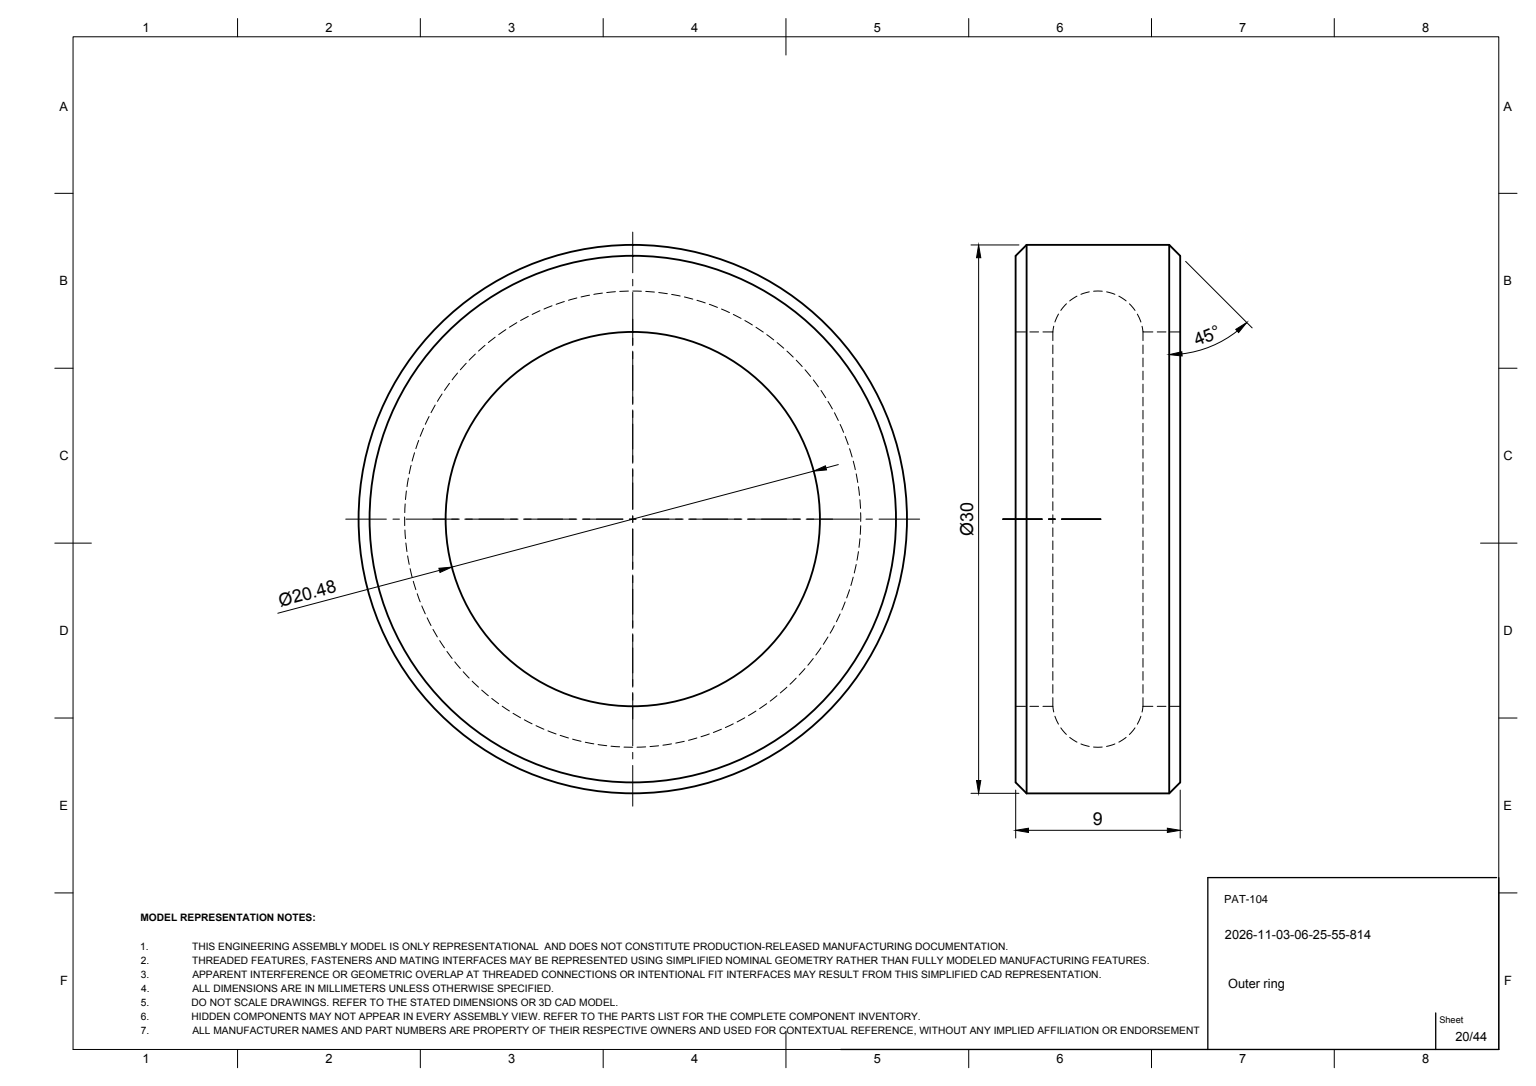
ISO-10303-21;
HEADER;
/* Generated by software containing ST-Developer
 * from STEP Tools, Inc. (www.steptools.com) 
 */

FILE_DESCRIPTION(
/* description */ ('Timing belt drive module 2 mm Pitch Timing 20T-40T'),

/* implementation_level */ '2;1');

FILE_NAME(
/* name */ 'Outer ring.step',
/* time_stamp */ '2026-10-28T03:25:12-07:00',
/* author */ (''),
/* organization */ (''),
/* preprocessor_version */ 'ST-DEVELOPER v20.2',
/* originating_system */ 'Autodesk Translation Framework v15.17.0.0',
/* authorisation */ '');

FILE_SCHEMA (('AUTOMOTIVE_DESIGN { 1 0 10303 214 3 1 1 }'));
ENDSEC;

DATA;
#10=MECHANICAL_DESIGN_GEOMETRIC_PRESENTATION_REPRESENTATION('',(#541),#17830);
#417=CONICAL_SURFACE('',#9909,1.47,0.785398163397449);
#418=CONICAL_SURFACE('',#9913,1.47,0.785398163397449);
#435=TOROIDAL_SURFACE('',#9898,1.,0.247676);
#455=SHAPE_REPRESENTATION_RELATIONSHIP('SRR','None',#18026,#498);
#498=ADVANCED_BREP_SHAPE_REPRESENTATION('',(#599),#17801);
#541=STYLED_ITEM('',(#18317),#599);
#599=MANIFOLD_SOLID_BREP('Body1',#8998);
#711=FACE_BOUND('',#1734,.T.);
#712=FACE_BOUND('',#1739,.T.);
#855=PLANE('',#9906);
#856=PLANE('',#9915);
#1136=FACE_OUTER_BOUND('',#1731,.T.);
#1137=FACE_OUTER_BOUND('',#1732,.T.);
#1138=FACE_OUTER_BOUND('',#1733,.T.);
#1139=FACE_OUTER_BOUND('',#1735,.T.);
#1140=FACE_OUTER_BOUND('',#1736,.T.);
#1141=FACE_OUTER_BOUND('',#1737,.T.);
#1142=FACE_OUTER_BOUND('',#1738,.T.);
#1143=FACE_OUTER_BOUND('',#1740,.T.);
#1731=EDGE_LOOP('',(#6573,#6574,#6575,#6576,#6577,#6578));
#1732=EDGE_LOOP('',(#6579,#6580,#6581,#6582,#6583));
#1733=EDGE_LOOP('',(#6584));
#1734=EDGE_LOOP('',(#6585));
#1735=EDGE_LOOP('',(#6586,#6587,#6588,#6589));
#1736=EDGE_LOOP('',(#6590,#6591,#6592,#6593));
#1737=EDGE_LOOP('',(#6594,#6595,#6596,#6597));
#1738=EDGE_LOOP('',(#6598));
#1739=EDGE_LOOP('',(#6599));
#1740=EDGE_LOOP('',(#6600,#6601,#6602,#6603,#6604));
#2327=CIRCLE('',#9899,1.023815);
#2328=CIRCLE('',#9900,1.023815);
#2329=CIRCLE('',#9901,0.247676);
#2330=CIRCLE('',#9902,1.023815);
#2331=CIRCLE('',#9903,1.023815);
#2332=CIRCLE('',#9905,1.023815);
#2333=CIRCLE('',#9907,1.44);
#2334=CIRCLE('',#9908,1.023815);
#2335=CIRCLE('',#9910,1.5);
#2336=CIRCLE('',#9912,1.5);
#2337=CIRCLE('',#9914,1.44);
#3003=LINE('',#14747,#3481);
#3004=LINE('',#14756,#3482);
#3005=LINE('',#14760,#3483);
#3006=LINE('',#14764,#3484);
#3007=LINE('',#14767,#3485);
#3481=VECTOR('',#11802,1.023815);
#3482=VECTOR('',#11813,1.47);
#3483=VECTOR('',#11818,1.5);
#3484=VECTOR('',#11823,1.47);
#3485=VECTOR('',#11828,1.023815);
#4012=VERTEX_POINT('',#14735);
#4013=VERTEX_POINT('',#14736);
#4014=VERTEX_POINT('',#14739);
#4015=VERTEX_POINT('',#14741);
#4016=VERTEX_POINT('',#14745);
#4017=VERTEX_POINT('',#14749);
#4018=VERTEX_POINT('',#14751);
#4019=VERTEX_POINT('',#14754);
#4020=VERTEX_POINT('',#14758);
#4021=VERTEX_POINT('',#14762);
#4969=EDGE_CURVE('',#4012,#4013,#2327,.T.);
#4970=EDGE_CURVE('',#4013,#4012,#2328,.T.);
#4971=EDGE_CURVE('',#4013,#4014,#2329,.T.);
#4972=EDGE_CURVE('',#4015,#4014,#2330,.T.);
#4973=EDGE_CURVE('',#4014,#4015,#2331,.T.);
#4974=EDGE_CURVE('',#4016,#4016,#2332,.T.);
#4975=EDGE_CURVE('',#4016,#4015,#3003,.T.);
#4976=EDGE_CURVE('',#4017,#4017,#2333,.T.);
#4977=EDGE_CURVE('',#4018,#4018,#2334,.T.);
#4978=EDGE_CURVE('',#4019,#4019,#2335,.T.);
#4979=EDGE_CURVE('',#4019,#4017,#3004,.T.);
#4980=EDGE_CURVE('',#4020,#4020,#2336,.T.);
#4981=EDGE_CURVE('',#4020,#4019,#3005,.T.);
#4982=EDGE_CURVE('',#4021,#4021,#2337,.T.);
#4983=EDGE_CURVE('',#4021,#4020,#3006,.T.);
#4984=EDGE_CURVE('',#4012,#4018,#3007,.T.);
#6573=ORIENTED_EDGE('',*,*,#4969,.F.);
#6574=ORIENTED_EDGE('',*,*,#4970,.F.);
#6575=ORIENTED_EDGE('',*,*,#4971,.T.);
#6576=ORIENTED_EDGE('',*,*,#4972,.F.);
#6577=ORIENTED_EDGE('',*,*,#4973,.F.);
#6578=ORIENTED_EDGE('',*,*,#4971,.F.);
#6579=ORIENTED_EDGE('',*,*,#4974,.T.);
#6580=ORIENTED_EDGE('',*,*,#4975,.T.);
#6581=ORIENTED_EDGE('',*,*,#4972,.T.);
#6582=ORIENTED_EDGE('',*,*,#4973,.T.);
#6583=ORIENTED_EDGE('',*,*,#4975,.F.);
#6584=ORIENTED_EDGE('',*,*,#4976,.F.);
#6585=ORIENTED_EDGE('',*,*,#4977,.T.);
#6586=ORIENTED_EDGE('',*,*,#4978,.F.);
#6587=ORIENTED_EDGE('',*,*,#4979,.T.);
#6588=ORIENTED_EDGE('',*,*,#4976,.T.);
#6589=ORIENTED_EDGE('',*,*,#4979,.F.);
#6590=ORIENTED_EDGE('',*,*,#4980,.F.);
#6591=ORIENTED_EDGE('',*,*,#4981,.T.);
#6592=ORIENTED_EDGE('',*,*,#4978,.T.);
#6593=ORIENTED_EDGE('',*,*,#4981,.F.);
#6594=ORIENTED_EDGE('',*,*,#4982,.F.);
#6595=ORIENTED_EDGE('',*,*,#4983,.T.);
#6596=ORIENTED_EDGE('',*,*,#4980,.T.);
#6597=ORIENTED_EDGE('',*,*,#4983,.F.);
#6598=ORIENTED_EDGE('',*,*,#4982,.T.);
#6599=ORIENTED_EDGE('',*,*,#4974,.F.);
#6600=ORIENTED_EDGE('',*,*,#4969,.T.);
#6601=ORIENTED_EDGE('',*,*,#4970,.T.);
#6602=ORIENTED_EDGE('',*,*,#4984,.T.);
#6603=ORIENTED_EDGE('',*,*,#4977,.F.);
#6604=ORIENTED_EDGE('',*,*,#4984,.F.);
#8270=CYLINDRICAL_SURFACE('',#9904,1.023815);
#8271=CYLINDRICAL_SURFACE('',#9911,1.5);
#8272=CYLINDRICAL_SURFACE('',#9916,1.023815);
#8634=ADVANCED_FACE('',(#1136),#435,.F.);
#8635=ADVANCED_FACE('',(#1137),#8270,.F.);
#8636=ADVANCED_FACE('',(#1138,#711),#855,.T.);
#8637=ADVANCED_FACE('',(#1139),#417,.T.);
#8638=ADVANCED_FACE('',(#1140),#8271,.T.);
#8639=ADVANCED_FACE('',(#1141),#418,.T.);
#8640=ADVANCED_FACE('',(#1142,#712),#856,.T.);
#8641=ADVANCED_FACE('',(#1143),#8272,.F.);
#8998=CLOSED_SHELL('',(#8634,#8635,#8636,#8637,#8638,#8639,#8640,#8641));
#9897=AXIS2_PLACEMENT_3D('',#14733,#11784,#11785);
#9898=AXIS2_PLACEMENT_3D('',#14734,#11786,#11787);
#9899=AXIS2_PLACEMENT_3D('',#14737,#11788,#11789);
#9900=AXIS2_PLACEMENT_3D('',#14738,#11790,#11791);
#9901=AXIS2_PLACEMENT_3D('',#14740,#11792,#11793);
#9902=AXIS2_PLACEMENT_3D('',#14742,#11794,#11795);
#9903=AXIS2_PLACEMENT_3D('',#14743,#11796,#11797);
#9904=AXIS2_PLACEMENT_3D('',#14744,#11798,#11799);
#9905=AXIS2_PLACEMENT_3D('',#14746,#11800,#11801);
#9906=AXIS2_PLACEMENT_3D('',#14748,#11803,#11804);
#9907=AXIS2_PLACEMENT_3D('',#14750,#11805,#11806);
#9908=AXIS2_PLACEMENT_3D('',#14752,#11807,#11808);
#9909=AXIS2_PLACEMENT_3D('',#14753,#11809,#11810);
#9910=AXIS2_PLACEMENT_3D('',#14755,#11811,#11812);
#9911=AXIS2_PLACEMENT_3D('',#14757,#11814,#11815);
#9912=AXIS2_PLACEMENT_3D('',#14759,#11816,#11817);
#9913=AXIS2_PLACEMENT_3D('',#14761,#11819,#11820);
#9914=AXIS2_PLACEMENT_3D('',#14763,#11821,#11822);
#9915=AXIS2_PLACEMENT_3D('',#14765,#11824,#11825);
#9916=AXIS2_PLACEMENT_3D('',#14766,#11826,#11827);
#11784=DIRECTION('axis',(0.,0.,1.));
#11785=DIRECTION('refdir',(1.,0.,0.));
#11786=DIRECTION('center_axis',(0.,-1.,0.));
#11787=DIRECTION('ref_axis',(0.,0.,-1.));
#11788=DIRECTION('center_axis',(0.,-1.,0.));
#11789=DIRECTION('ref_axis',(1.,0.,0.));
#11790=DIRECTION('center_axis',(0.,-1.,0.));
#11791=DIRECTION('ref_axis',(1.,0.,0.));
#11792=DIRECTION('center_axis',(1.,0.,1.22464679914735E-16));
#11793=DIRECTION('ref_axis',(-1.22464679914735E-16,0.,1.));
#11794=DIRECTION('center_axis',(0.,1.,0.));
#11795=DIRECTION('ref_axis',(1.,0.,0.));
#11796=DIRECTION('center_axis',(0.,1.,0.));
#11797=DIRECTION('ref_axis',(1.,0.,0.));
#11798=DIRECTION('center_axis',(0.,-1.,0.));
#11799=DIRECTION('ref_axis',(1.,0.,0.));
#11800=DIRECTION('center_axis',(0.,-1.,0.));
#11801=DIRECTION('ref_axis',(1.,0.,0.));
#11802=DIRECTION('',(0.,1.,0.));
#11803=DIRECTION('center_axis',(0.,1.,0.));
#11804=DIRECTION('ref_axis',(0.,0.,1.));
#11805=DIRECTION('center_axis',(0.,-1.,0.));
#11806=DIRECTION('ref_axis',(1.,0.,0.));
#11807=DIRECTION('center_axis',(0.,-1.,0.));
#11808=DIRECTION('ref_axis',(1.,0.,0.));
#11809=DIRECTION('center_axis',(0.,-1.,0.));
#11810=DIRECTION('ref_axis',(1.,0.,0.));
#11811=DIRECTION('center_axis',(0.,-1.,0.));
#11812=DIRECTION('ref_axis',(1.,0.,0.));
#11813=DIRECTION('',(0.707106781186548,0.707106781186547,8.65956056235494E-17));
#11814=DIRECTION('center_axis',(0.,-1.,0.));
#11815=DIRECTION('ref_axis',(1.,0.,0.));
#11816=DIRECTION('center_axis',(0.,-1.,0.));
#11817=DIRECTION('ref_axis',(1.,0.,0.));
#11818=DIRECTION('',(0.,1.,0.));
#11819=DIRECTION('center_axis',(0.,1.,0.));
#11820=DIRECTION('ref_axis',(1.,0.,0.));
#11821=DIRECTION('center_axis',(0.,-1.,0.));
#11822=DIRECTION('ref_axis',(1.,0.,0.));
#11823=DIRECTION('',(-0.707106781186548,0.707106781186547,-8.65956056235494E-17));
#11824=DIRECTION('center_axis',(0.,-1.,0.));
#11825=DIRECTION('ref_axis',(0.,0.,-1.));
#11826=DIRECTION('center_axis',(0.,-1.,0.));
#11827=DIRECTION('ref_axis',(1.,0.,0.));
#11828=DIRECTION('',(0.,1.,0.));
#14733=CARTESIAN_POINT('',(0.,0.,0.));
#14734=CARTESIAN_POINT('Origin',(0.,0.,0.));
#14735=CARTESIAN_POINT('',(-1.023815,0.246528389340863,-1.25381176266905E-16));
#14736=CARTESIAN_POINT('',(-1.25381176266905E-16,0.246528389340863,1.023815));
#14737=CARTESIAN_POINT('Origin',(0.,0.246528389340863,0.));
#14738=CARTESIAN_POINT('Origin',(0.,0.246528389340863,0.));
#14739=CARTESIAN_POINT('',(-1.25381176266905E-16,-0.246528389340863,1.023815));
#14740=CARTESIAN_POINT('Origin',(-1.22464679914735E-16,0.,1.));
#14741=CARTESIAN_POINT('',(-1.023815,-0.246528389340863,1.25381176266905E-16));
#14742=CARTESIAN_POINT('Origin',(0.,-0.246528389340863,0.));
#14743=CARTESIAN_POINT('Origin',(0.,-0.246528389340863,0.));
#14744=CARTESIAN_POINT('Origin',(0.,0.,0.));
#14745=CARTESIAN_POINT('',(-1.023815,-0.45,-1.25381176266905E-16));
#14746=CARTESIAN_POINT('Origin',(0.,-0.45,0.));
#14747=CARTESIAN_POINT('',(-1.023815,0.,-1.25381176266905E-16));
#14748=CARTESIAN_POINT('Origin',(1.44,0.45,0.));
#14749=CARTESIAN_POINT('',(-1.44,0.45,-1.76349139077219E-16));
#14750=CARTESIAN_POINT('Origin',(0.,0.45,0.));
#14751=CARTESIAN_POINT('',(-1.023815,0.45,-1.25381176266905E-16));
#14752=CARTESIAN_POINT('Origin',(0.,0.45,0.));
#14753=CARTESIAN_POINT('Origin',(0.,0.42,0.));
#14754=CARTESIAN_POINT('',(-1.5,0.39,-1.83697019872103E-16));
#14755=CARTESIAN_POINT('Origin',(0.,0.39,0.));
#14756=CARTESIAN_POINT('',(-1.47,0.42,-1.80023079474661E-16));
#14757=CARTESIAN_POINT('Origin',(0.,0.,0.));
#14758=CARTESIAN_POINT('',(-1.5,-0.39,-1.83697019872103E-16));
#14759=CARTESIAN_POINT('Origin',(0.,-0.39,0.));
#14760=CARTESIAN_POINT('',(-1.5,0.,-1.83697019872103E-16));
#14761=CARTESIAN_POINT('Origin',(0.,-0.42,0.));
#14762=CARTESIAN_POINT('',(-1.44,-0.45,-1.76349139077219E-16));
#14763=CARTESIAN_POINT('Origin',(0.,-0.45,0.));
#14764=CARTESIAN_POINT('',(-1.47,-0.42,-1.80023079474661E-16));
#14765=CARTESIAN_POINT('Origin',(1.023815,-0.45,0.));
#14766=CARTESIAN_POINT('Origin',(0.,0.,0.));
#14767=CARTESIAN_POINT('',(-1.023815,0.,-1.25381176266905E-16));
#17751=UNCERTAINTY_MEASURE_WITH_UNIT(LENGTH_MEASURE(0.001),#17831,
'DISTANCE_ACCURACY_VALUE',
'Maximum model space distance between geometric entities at asserted c
onnectivities');
#17780=UNCERTAINTY_MEASURE_WITH_UNIT(LENGTH_MEASURE(0.001),#17831,
'DISTANCE_ACCURACY_VALUE',
'Maximum model space distance between geometric entities at asserted c
onnectivities');
#17801=(
GEOMETRIC_REPRESENTATION_CONTEXT(3)
GLOBAL_UNCERTAINTY_ASSIGNED_CONTEXT((#17751))
GLOBAL_UNIT_ASSIGNED_CONTEXT((#17831,#17833,#17834))
REPRESENTATION_CONTEXT('','3D')
);
#17830=(
GEOMETRIC_REPRESENTATION_CONTEXT(3)
GLOBAL_UNCERTAINTY_ASSIGNED_CONTEXT((#17780))
GLOBAL_UNIT_ASSIGNED_CONTEXT((#17831,#17833,#17834))
REPRESENTATION_CONTEXT('','3D')
);
#17831=(
LENGTH_UNIT()
NAMED_UNIT(*)
SI_UNIT(.CENTI.,.METRE.)
);
#17833=(
NAMED_UNIT(*)
PLANE_ANGLE_UNIT()
SI_UNIT($,.RADIAN.)
);
#17834=(
NAMED_UNIT(*)
SI_UNIT($,.STERADIAN.)
SOLID_ANGLE_UNIT()
);
#17855=SHAPE_DEFINITION_REPRESENTATION(#17904,#18026);
#17904=PRODUCT_DEFINITION_SHAPE('',$,#18076);
#18026=SHAPE_REPRESENTATION('',(#9897),#17801);
#18055=PRODUCT_DEFINITION_CONTEXT('part definition',#18204,'design');
#18076=PRODUCT_DEFINITION('Outer ring','Outer ring',#18125,#18055);
#18125=PRODUCT_DEFINITION_FORMATION('',$,#18226);
#18204=APPLICATION_CONTEXT(
'Core Data for Automotive Mechanical Design Process');
#18205=PRODUCT_CONTEXT('part definition',#18204,'mechanical');
#18226=PRODUCT('Outer ring','Outer ring','Outer ring',(#18205));
#18311=COLOUR_RGB('Grey',0.48,0.52,0.57);
#18312=FILL_AREA_STYLE_COLOUR('',#18311);
#18313=FILL_AREA_STYLE('',(#18312));
#18314=SURFACE_STYLE_FILL_AREA(#18313);
#18315=SURFACE_SIDE_STYLE('',(#18314));
#18316=SURFACE_STYLE_USAGE(.BOTH.,#18315);
#18317=PRESENTATION_STYLE_ASSIGNMENT((#18316));
ENDSEC;
END-ISO-10303-21;
